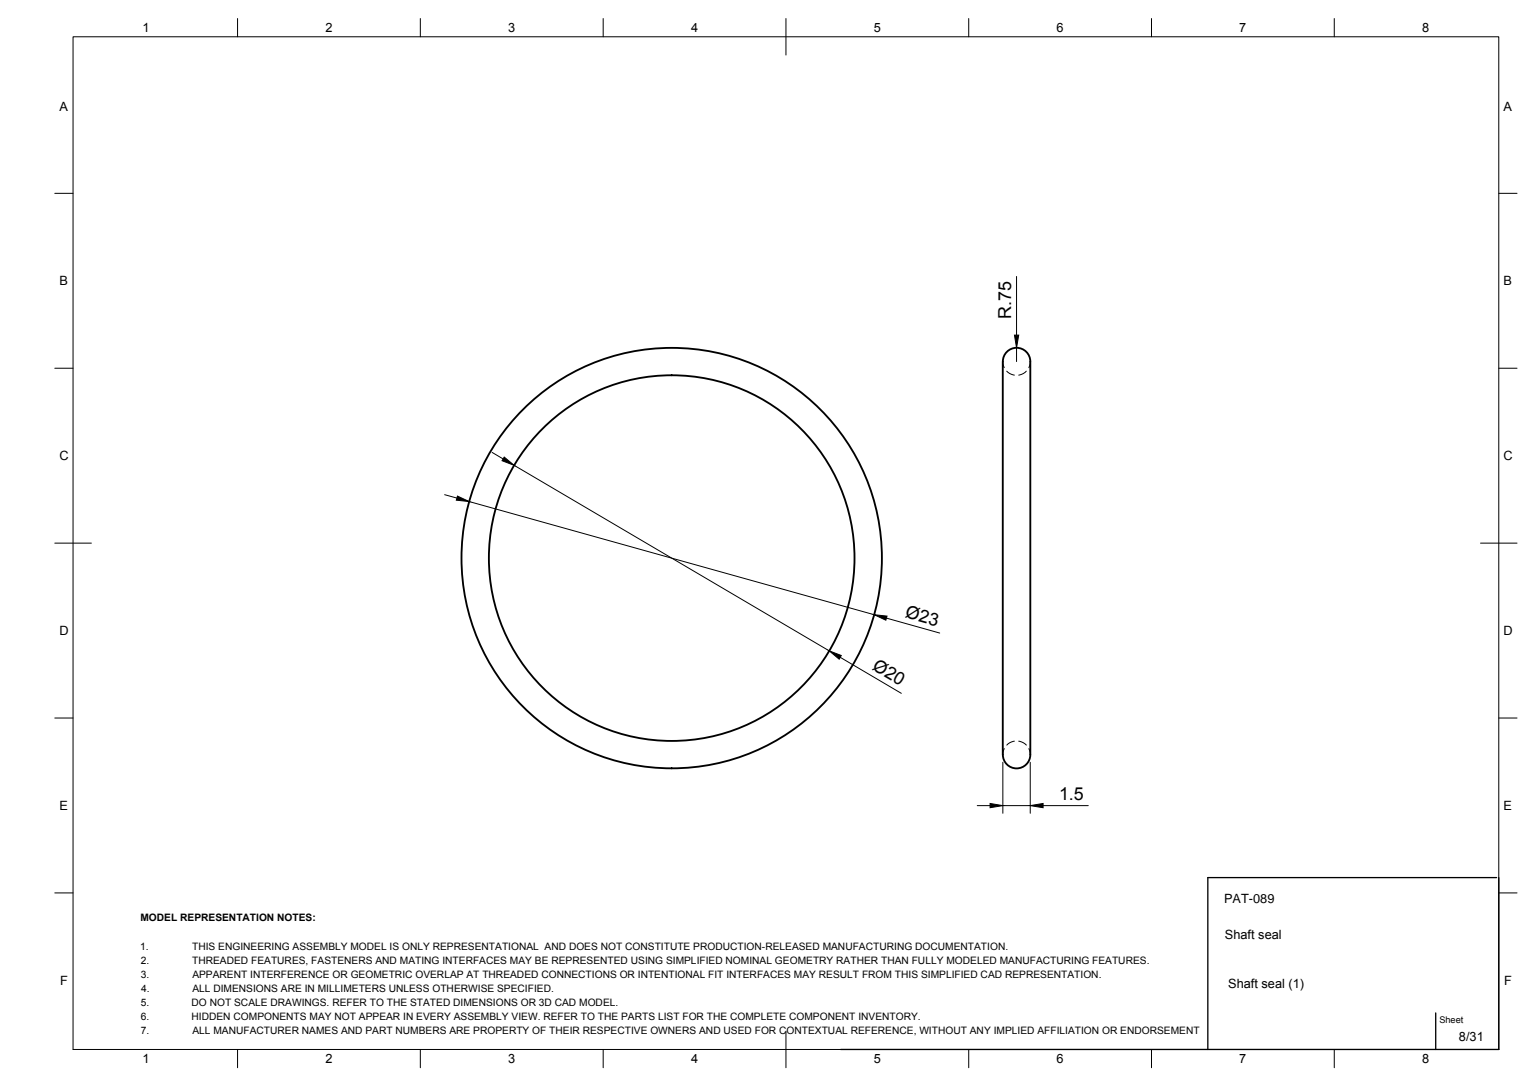
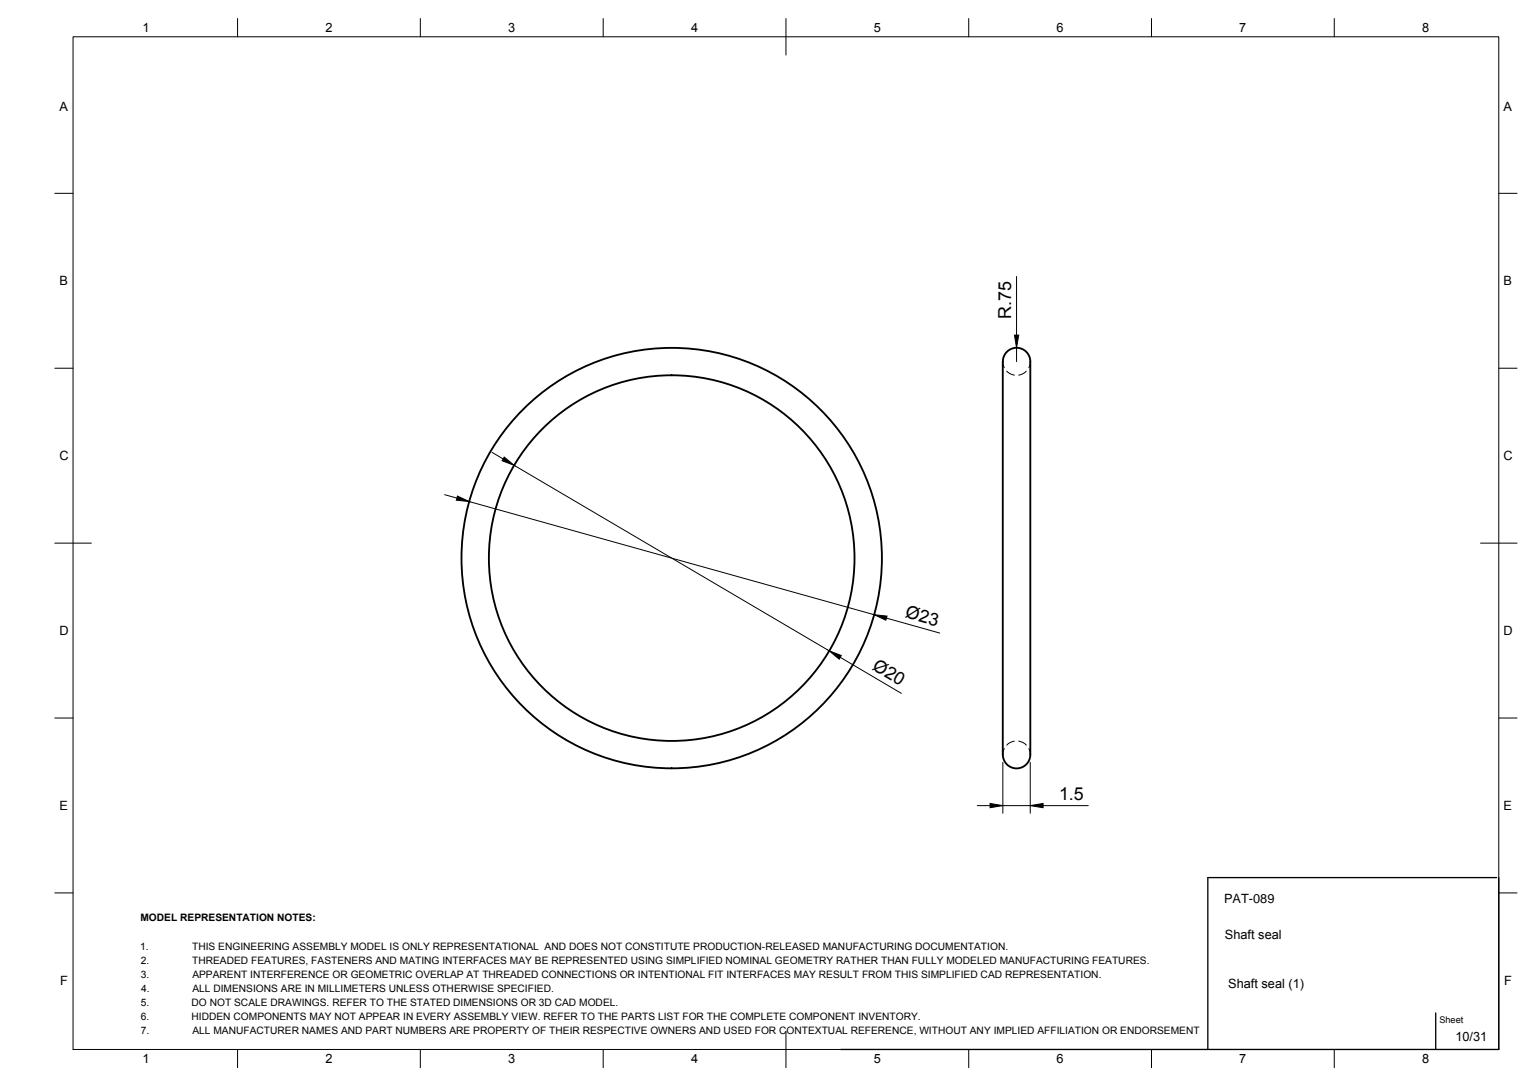
ISO-10303-21;
HEADER;
/* Generated by software containing ST-Developer
 * from STEP Tools, Inc. (www.steptools.com) 
 */

FILE_DESCRIPTION(
/* description */ ('Rotary union on bearing shaft'),
/* implementation_level */ '2;1');

FILE_NAME(
/* name */ 'Shaft seal (1).step',
/* time_stamp */ '2026-10-28T03:24:01-07:00',
/* author */ (''),
/* organization */ (''),
/* preprocessor_version */ 'ST-DEVELOPER v20.2',
/* originating_system */ 'Autodesk Translation Framework v15.17.0.0',
/* authorisation */ '');

FILE_SCHEMA (('AUTOMOTIVE_DESIGN { 1 0 10303 214 3 1 1 }'));
ENDSEC;

DATA;
#10=MECHANICAL_DESIGN_GEOMETRIC_PRESENTATION_REPRESENTATION('',(#318),#9448);
#222=TOROIDAL_SURFACE('',#5344,1.075,0.075);
#264=SHAPE_REPRESENTATION_RELATIONSHIP('SRR','None',#9564,#291);
#291=ADVANCED_BREP_SHAPE_REPRESENTATION('',(#353),#9424);
#318=STYLED_ITEM('',(#9785),#353);
#353=MANIFOLD_SOLID_BREP('Body1',#4873);
#726=FACE_OUTER_BOUND('',#1063,.T.);
#1063=EDGE_LOOP('',(#3549,#3550,#3551,#3552));
#2063=CIRCLE('',#5345,0.075);
#2064=CIRCLE('',#5346,1.);
#2346=VERTEX_POINT('',#7777);
#2802=EDGE_CURVE('',#2346,#2346,#2063,.T.);
#2803=EDGE_CURVE('',#2346,#2346,#2064,.T.);
#3549=ORIENTED_EDGE('',*,*,#2802,.F.);
#3550=ORIENTED_EDGE('',*,*,#2803,.T.);
#3551=ORIENTED_EDGE('',*,*,#2802,.T.);
#3552=ORIENTED_EDGE('',*,*,#2803,.F.);
#4639=ADVANCED_FACE('',(#726),#222,.T.);
#4873=CLOSED_SHELL('',(#4639));
#5343=AXIS2_PLACEMENT_3D('',#7775,#6181,#6182);
#5344=AXIS2_PLACEMENT_3D('',#7776,#6183,#6184);
#5345=AXIS2_PLACEMENT_3D('',#7778,#6185,#6186);
#5346=AXIS2_PLACEMENT_3D('',#7779,#6187,#6188);
#6181=DIRECTION('axis',(0.,0.,1.));
#6182=DIRECTION('refdir',(1.,0.,0.));
#6183=DIRECTION('center_axis',(0.,-1.,0.));
#6184=DIRECTION('ref_axis',(0.,0.,-1.));
#6185=DIRECTION('center_axis',(-1.,0.,-1.22464679914735E-16));
#6186=DIRECTION('ref_axis',(-1.22464679914735E-16,0.,1.));
#6187=DIRECTION('center_axis',(0.,1.,0.));
#6188=DIRECTION('ref_axis',(0.,0.,-1.));
#7775=CARTESIAN_POINT('',(0.,0.,0.));
#7776=CARTESIAN_POINT('Origin',(0.,3.95,4.5));
#7777=CARTESIAN_POINT('',(-1.22464679914735E-16,3.95,5.5));
#7778=CARTESIAN_POINT('Origin',(-1.3164953090834E-16,3.95,5.575));
#7779=CARTESIAN_POINT('Origin',(0.,3.95,4.5));
#9392=UNCERTAINTY_MEASURE_WITH_UNIT(LENGTH_MEASURE(0.001),#9449,
'DISTANCE_ACCURACY_VALUE',
'Maximum model space distance between geometric entities at asserted c
onnectivities');
#9416=UNCERTAINTY_MEASURE_WITH_UNIT(LENGTH_MEASURE(0.001),#9449,
'DISTANCE_ACCURACY_VALUE',
'Maximum model space distance between geometric entities at asserted c
onnectivities');
#9424=(
GEOMETRIC_REPRESENTATION_CONTEXT(3)
GLOBAL_UNCERTAINTY_ASSIGNED_CONTEXT((#9392))
GLOBAL_UNIT_ASSIGNED_CONTEXT((#9449,#9451,#9452))
REPRESENTATION_CONTEXT('','3D')
);
#9448=(
GEOMETRIC_REPRESENTATION_CONTEXT(3)
GLOBAL_UNCERTAINTY_ASSIGNED_CONTEXT((#9416))
GLOBAL_UNIT_ASSIGNED_CONTEXT((#9449,#9451,#9452))
REPRESENTATION_CONTEXT('','3D')
);
#9449=(
LENGTH_UNIT()
NAMED_UNIT(*)
SI_UNIT(.CENTI.,.METRE.)
);
#9451=(
NAMED_UNIT(*)
PLANE_ANGLE_UNIT()
SI_UNIT($,.RADIAN.)
);
#9452=(
NAMED_UNIT(*)
SI_UNIT($,.STERADIAN.)
SOLID_ANGLE_UNIT()
);
#9460=SHAPE_DEFINITION_REPRESENTATION(#9491,#9564);
#9491=PRODUCT_DEFINITION_SHAPE('',$,#9596);
#9564=SHAPE_REPRESENTATION('',(#5343),#9424);
#9588=PRODUCT_DEFINITION_CONTEXT('part definition',#9683,'design');
#9596=PRODUCT_DEFINITION('Shaft seal (1)','Shaft seal (1)',#9627,#9588);
#9627=PRODUCT_DEFINITION_FORMATION('',$,#9692);
#9683=APPLICATION_CONTEXT(
'Core Data for Automotive Mechanical Design Process');
#9684=PRODUCT_CONTEXT('part definition',#9683,'mechanical');
#9692=PRODUCT('Shaft seal (1)','Shaft seal (1)','Shaft seal (1)',(#9684));
#9779=COLOUR_RGB('Black',0.12,0.14,0.17);
#9780=FILL_AREA_STYLE_COLOUR('',#9779);
#9781=FILL_AREA_STYLE('',(#9780));
#9782=SURFACE_STYLE_FILL_AREA(#9781);
#9783=SURFACE_SIDE_STYLE('',(#9782));
#9784=SURFACE_STYLE_USAGE(.BOTH.,#9783);
#9785=PRESENTATION_STYLE_ASSIGNMENT((#9784));
ENDSEC;
END-ISO-10303-21;
